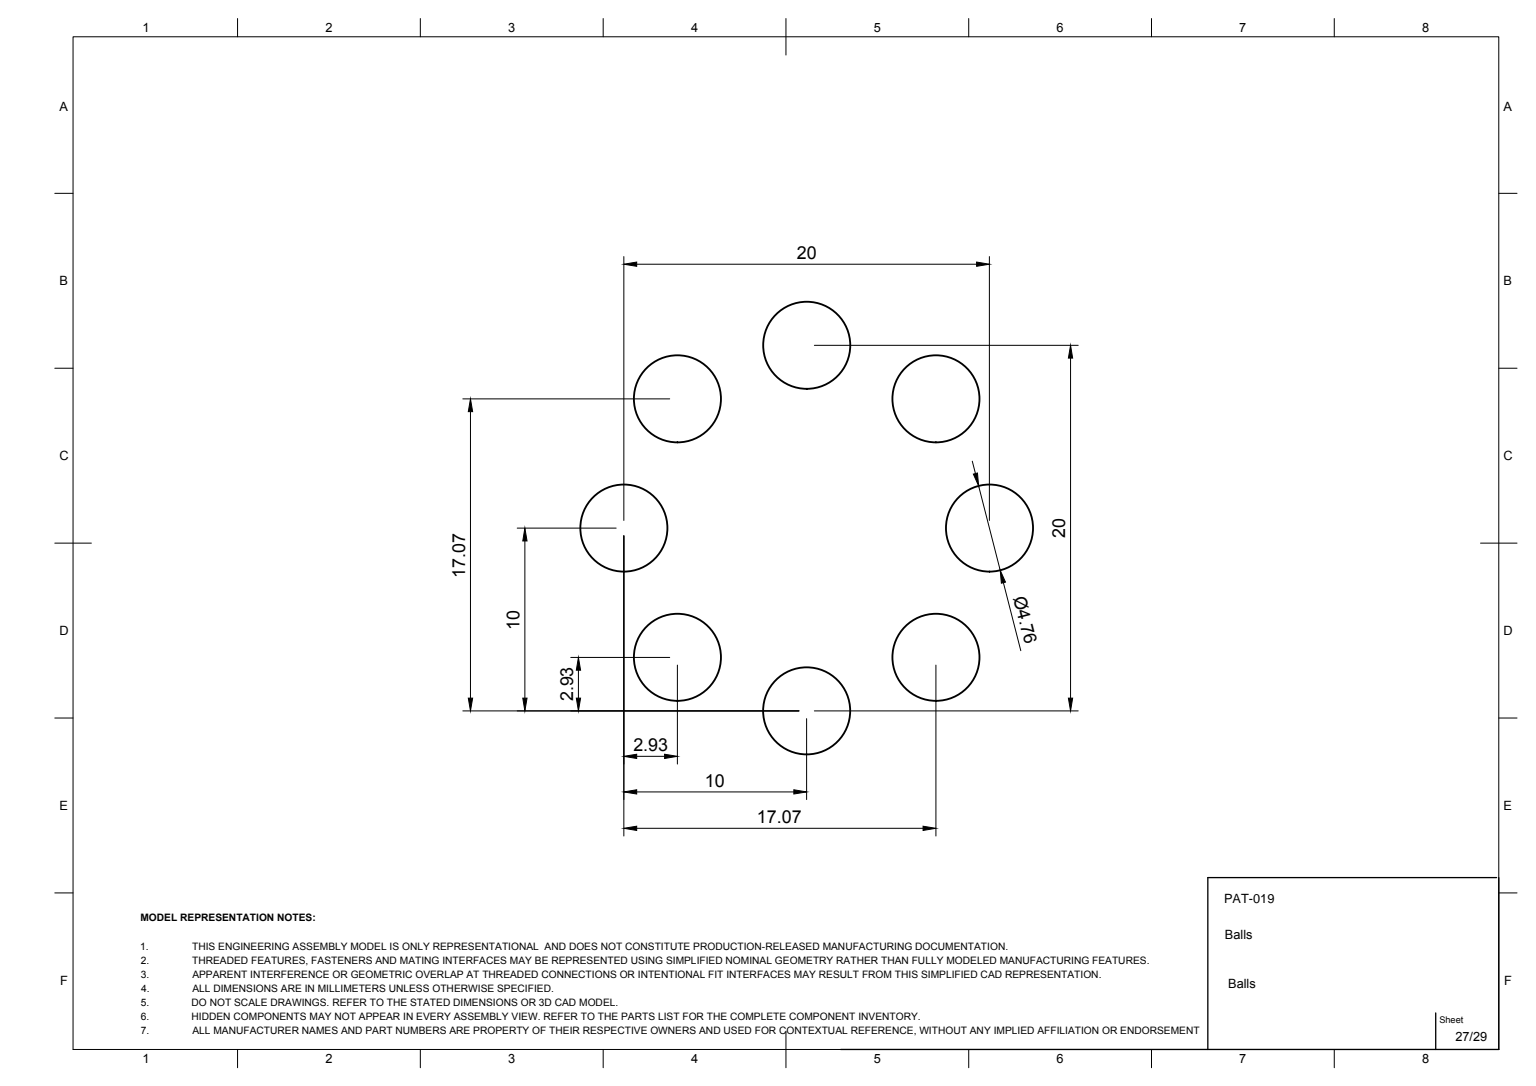
ISO-10303-21;
HEADER;
/* Generated by software containing ST-Developer
 * from STEP Tools, Inc. (www.steptools.com) 
 */

FILE_DESCRIPTION(
/* description */ ('Caster wheel assembly'),
/* implementation_level */ '2;1');

FILE_NAME(
/* name */ 'Balls.step',
/* time_stamp */ '2026-10-28T03:23:56-07:00',
/* author */ (''),
/* organization */ (''),
/* preprocessor_version */ 'ST-DEVELOPER v20.2',
/* originating_system */ 'Autodesk Translation Framework v15.17.0.0',
/* authorisation */ '');

FILE_SCHEMA (('AUTOMOTIVE_DESIGN { 1 0 10303 214 3 1 1 }'));
ENDSEC;

DATA;
#10=MECHANICAL_DESIGN_GEOMETRIC_PRESENTATION_REPRESENTATION('',(#241,#242,#243,#244,#245,#246,#247,#248),#5385);
#29=SPHERICAL_SURFACE('',#3204,0.23815);
#30=SPHERICAL_SURFACE('',#3206,0.23815);
#31=SPHERICAL_SURFACE('',#3208,0.23815);
#32=SPHERICAL_SURFACE('',#3210,0.23815);
#33=SPHERICAL_SURFACE('',#3212,0.23815);
#34=SPHERICAL_SURFACE('',#3214,0.23815);
#35=SPHERICAL_SURFACE('',#3216,0.23815);
#36=SPHERICAL_SURFACE('',#3218,0.23815);
#197=SHAPE_REPRESENTATION_RELATIONSHIP('SRR','None',#5495,#219);
#219=ADVANCED_BREP_SHAPE_REPRESENTATION('',(#270,#271,#272,#273,#274,#275,
#276,#277),#5382);
#241=STYLED_ITEM('',(#5672),#270);
#242=STYLED_ITEM('',(#5672),#271);
#243=STYLED_ITEM('',(#5672),#272);
#244=STYLED_ITEM('',(#5672),#273);
#245=STYLED_ITEM('',(#5672),#274);
#246=STYLED_ITEM('',(#5672),#275);
#247=STYLED_ITEM('',(#5672),#276);
#248=STYLED_ITEM('',(#5672),#277);
#270=MANIFOLD_SOLID_BREP('Body1',#2669);
#271=MANIFOLD_SOLID_BREP('Body2',#2670);
#272=MANIFOLD_SOLID_BREP('Body3',#2671);
#273=MANIFOLD_SOLID_BREP('Body4',#2672);
#274=MANIFOLD_SOLID_BREP('Body5',#2673);
#275=MANIFOLD_SOLID_BREP('Body6',#2674);
#276=MANIFOLD_SOLID_BREP('Body7',#2675);
#277=MANIFOLD_SOLID_BREP('Body8',#2676);
#554=FACE_OUTER_BOUND('',#769,.T.);
#555=FACE_OUTER_BOUND('',#770,.T.);
#556=FACE_OUTER_BOUND('',#771,.T.);
#557=FACE_OUTER_BOUND('',#772,.T.);
#558=FACE_OUTER_BOUND('',#773,.T.);
#559=FACE_OUTER_BOUND('',#774,.T.);
#560=FACE_OUTER_BOUND('',#775,.T.);
#561=FACE_OUTER_BOUND('',#776,.T.);
#769=EDGE_LOOP('',(#2280,#2281));
#770=EDGE_LOOP('',(#2282,#2283));
#771=EDGE_LOOP('',(#2284,#2285));
#772=EDGE_LOOP('',(#2286,#2287));
#773=EDGE_LOOP('',(#2288,#2289));
#774=EDGE_LOOP('',(#2290,#2291));
#775=EDGE_LOOP('',(#2292,#2293));
#776=EDGE_LOOP('',(#2294,#2295));
#1186=CIRCLE('',#3205,0.23815);
#1187=CIRCLE('',#3207,0.23815);
#1188=CIRCLE('',#3209,0.23815);
#1189=CIRCLE('',#3211,0.23815);
#1190=CIRCLE('',#3213,0.23815);
#1191=CIRCLE('',#3215,0.23815);
#1192=CIRCLE('',#3217,0.23815);
#1193=CIRCLE('',#3219,0.23815);
#1399=VERTEX_POINT('',#4809);
#1400=VERTEX_POINT('',#4810);
#1401=VERTEX_POINT('',#4813);
#1402=VERTEX_POINT('',#4814);
#1403=VERTEX_POINT('',#4817);
#1404=VERTEX_POINT('',#4818);
#1405=VERTEX_POINT('',#4821);
#1406=VERTEX_POINT('',#4822);
#1407=VERTEX_POINT('',#4825);
#1408=VERTEX_POINT('',#4826);
#1409=VERTEX_POINT('',#4829);
#1410=VERTEX_POINT('',#4830);
#1411=VERTEX_POINT('',#4833);
#1412=VERTEX_POINT('',#4834);
#1413=VERTEX_POINT('',#4837);
#1414=VERTEX_POINT('',#4838);
#1708=EDGE_CURVE('',#1399,#1400,#1186,.T.);
#1709=EDGE_CURVE('',#1401,#1402,#1187,.T.);
#1710=EDGE_CURVE('',#1403,#1404,#1188,.T.);
#1711=EDGE_CURVE('',#1405,#1406,#1189,.T.);
#1712=EDGE_CURVE('',#1407,#1408,#1190,.T.);
#1713=EDGE_CURVE('',#1409,#1410,#1191,.T.);
#1714=EDGE_CURVE('',#1411,#1412,#1192,.T.);
#1715=EDGE_CURVE('',#1413,#1414,#1193,.T.);
#2280=ORIENTED_EDGE('',*,*,#1708,.T.);
#2281=ORIENTED_EDGE('',*,*,#1708,.F.);
#2282=ORIENTED_EDGE('',*,*,#1709,.T.);
#2283=ORIENTED_EDGE('',*,*,#1709,.F.);
#2284=ORIENTED_EDGE('',*,*,#1710,.T.);
#2285=ORIENTED_EDGE('',*,*,#1710,.F.);
#2286=ORIENTED_EDGE('',*,*,#1711,.T.);
#2287=ORIENTED_EDGE('',*,*,#1711,.F.);
#2288=ORIENTED_EDGE('',*,*,#1712,.T.);
#2289=ORIENTED_EDGE('',*,*,#1712,.F.);
#2290=ORIENTED_EDGE('',*,*,#1713,.T.);
#2291=ORIENTED_EDGE('',*,*,#1713,.F.);
#2292=ORIENTED_EDGE('',*,*,#1714,.T.);
#2293=ORIENTED_EDGE('',*,*,#1714,.F.);
#2294=ORIENTED_EDGE('',*,*,#1715,.T.);
#2295=ORIENTED_EDGE('',*,*,#1715,.F.);
#2614=ADVANCED_FACE('',(#554),#29,.T.);
#2615=ADVANCED_FACE('',(#555),#30,.T.);
#2616=ADVANCED_FACE('',(#556),#31,.T.);
#2617=ADVANCED_FACE('',(#557),#32,.T.);
#2618=ADVANCED_FACE('',(#558),#33,.T.);
#2619=ADVANCED_FACE('',(#559),#34,.T.);
#2620=ADVANCED_FACE('',(#560),#35,.T.);
#2621=ADVANCED_FACE('',(#561),#36,.T.);
#2669=CLOSED_SHELL('',(#2614));
#2670=CLOSED_SHELL('',(#2615));
#2671=CLOSED_SHELL('',(#2616));
#2672=CLOSED_SHELL('',(#2617));
#2673=CLOSED_SHELL('',(#2618));
#2674=CLOSED_SHELL('',(#2619));
#2675=CLOSED_SHELL('',(#2620));
#2676=CLOSED_SHELL('',(#2621));
#3203=AXIS2_PLACEMENT_3D('',#4807,#3992,#3993);
#3204=AXIS2_PLACEMENT_3D('',#4808,#3994,#3995);
#3205=AXIS2_PLACEMENT_3D('',#4811,#3996,#3997);
#3206=AXIS2_PLACEMENT_3D('',#4812,#3998,#3999);
#3207=AXIS2_PLACEMENT_3D('',#4815,#4000,#4001);
#3208=AXIS2_PLACEMENT_3D('',#4816,#4002,#4003);
#3209=AXIS2_PLACEMENT_3D('',#4819,#4004,#4005);
#3210=AXIS2_PLACEMENT_3D('',#4820,#4006,#4007);
#3211=AXIS2_PLACEMENT_3D('',#4823,#4008,#4009);
#3212=AXIS2_PLACEMENT_3D('',#4824,#4010,#4011);
#3213=AXIS2_PLACEMENT_3D('',#4827,#4012,#4013);
#3214=AXIS2_PLACEMENT_3D('',#4828,#4014,#4015);
#3215=AXIS2_PLACEMENT_3D('',#4831,#4016,#4017);
#3216=AXIS2_PLACEMENT_3D('',#4832,#4018,#4019);
#3217=AXIS2_PLACEMENT_3D('',#4835,#4020,#4021);
#3218=AXIS2_PLACEMENT_3D('',#4836,#4022,#4023);
#3219=AXIS2_PLACEMENT_3D('',#4839,#4024,#4025);
#3992=DIRECTION('axis',(0.,0.,1.));
#3993=DIRECTION('refdir',(1.,0.,0.));
#3994=DIRECTION('center_axis',(0.,0.,1.));
#3995=DIRECTION('ref_axis',(1.,0.,0.));
#3996=DIRECTION('center_axis',(1.22464679914735E-16,-1.,0.));
#3997=DIRECTION('ref_axis',(-1.,-1.22464679914735E-16,0.));
#3998=DIRECTION('center_axis',(0.707106781186548,0.,0.707106781186548));
#3999=DIRECTION('ref_axis',(0.707106781186548,0.,-0.707106781186548));
#4000=DIRECTION('center_axis',(8.65956056235494E-17,-1.,-8.65956056235493E-17));
#4001=DIRECTION('ref_axis',(-0.707106781186547,-1.22464679914735E-16,0.707106781186547));
#4002=DIRECTION('center_axis',(1.,0.,0.));
#4003=DIRECTION('ref_axis',(6.12323399573676E-17,0.,-1.));
#4004=DIRECTION('center_axis',(7.49879891330929E-33,-1.,-1.22464679914735E-16));
#4005=DIRECTION('ref_axis',(-6.12323399573676E-17,-1.22464679914735E-16,
1.));
#4006=DIRECTION('center_axis',(0.707106781186548,0.,-0.707106781186548));
#4007=DIRECTION('ref_axis',(-0.707106781186548,0.,-0.707106781186548));
#4008=DIRECTION('center_axis',(-8.65956056235493E-17,-1.,-8.65956056235494E-17));
#4009=DIRECTION('ref_axis',(0.707106781186547,-1.22464679914735E-16,0.707106781186547));
#4010=DIRECTION('center_axis',(0.,0.,-1.));
#4011=DIRECTION('ref_axis',(-1.,0.,-1.22464679914735E-16));
#4012=DIRECTION('center_axis',(-1.22464679914735E-16,-1.,-1.49975978266186E-32));
#4013=DIRECTION('ref_axis',(1.,-1.22464679914735E-16,1.22464679914735E-16));
#4014=DIRECTION('center_axis',(-0.707106781186547,0.,-0.707106781186548));
#4015=DIRECTION('ref_axis',(-0.707106781186548,0.,0.707106781186547));
#4016=DIRECTION('center_axis',(-8.65956056235493E-17,-1.,8.65956056235493E-17));
#4017=DIRECTION('ref_axis',(0.707106781186548,-1.22464679914735E-16,-0.707106781186547));
#4018=DIRECTION('center_axis',(-1.,0.,0.));
#4019=DIRECTION('ref_axis',(-1.83697019872103E-16,0.,1.));
#4020=DIRECTION('center_axis',(-2.24963967399279E-32,-1.,1.22464679914735E-16));
#4021=DIRECTION('ref_axis',(1.83697019872103E-16,-1.22464679914735E-16,
-1.));
#4022=DIRECTION('center_axis',(-0.707106781186548,0.,0.707106781186548));
#4023=DIRECTION('ref_axis',(0.707106781186547,0.,0.707106781186548));
#4024=DIRECTION('center_axis',(8.65956056235493E-17,-1.,8.65956056235493E-17));
#4025=DIRECTION('ref_axis',(-0.707106781186547,-1.22464679914735E-16,-0.707106781186548));
#4807=CARTESIAN_POINT('',(0.,0.,0.));
#4808=CARTESIAN_POINT('Origin',(1.,0.,0.));
#4809=CARTESIAN_POINT('',(1.,-1.78583896120461E-33,0.23815));
#4810=CARTESIAN_POINT('',(1.,-1.78583896120461E-33,-0.23815));
#4811=CARTESIAN_POINT('Origin',(1.,0.,0.));
#4812=CARTESIAN_POINT('Origin',(0.707106781186548,0.,-0.707106781186547));
#4813=CARTESIAN_POINT('',(0.875504261126124,-1.78583896120461E-33,-0.538709301246971));
#4814=CARTESIAN_POINT('',(0.538709301246971,-1.78583896120461E-33,-0.875504261126124));
#4815=CARTESIAN_POINT('Origin',(0.707106781186548,0.,-0.707106781186547));
#4816=CARTESIAN_POINT('Origin',(6.12323399573677E-17,0.,-1.));
#4817=CARTESIAN_POINT('',(0.23815,-1.78583896120461E-33,-1.));
#4818=CARTESIAN_POINT('',(-0.23815,-1.78583896120461E-33,-1.));
#4819=CARTESIAN_POINT('Origin',(6.12323399573677E-17,0.,-1.));
#4820=CARTESIAN_POINT('Origin',(-0.707106781186547,0.,-0.707106781186548));
#4821=CARTESIAN_POINT('',(-0.538709301246971,-1.78583896120461E-33,-0.875504261126124));
#4822=CARTESIAN_POINT('',(-0.875504261126124,-1.78583896120461E-33,-0.538709301246971));
#4823=CARTESIAN_POINT('Origin',(-0.707106781186547,0.,-0.707106781186548));
#4824=CARTESIAN_POINT('Origin',(-1.,0.,-1.22464679914735E-16));
#4825=CARTESIAN_POINT('',(-1.,-1.78583896120461E-33,-0.23815));
#4826=CARTESIAN_POINT('',(-1.,-1.78583896120461E-33,0.23815));
#4827=CARTESIAN_POINT('Origin',(-1.,0.,-1.22464679914735E-16));
#4828=CARTESIAN_POINT('Origin',(-0.707106781186548,0.,0.707106781186547));
#4829=CARTESIAN_POINT('',(-0.875504261126124,-7.94881478324376E-33,0.538709301246971));
#4830=CARTESIAN_POINT('',(-0.538709301246971,4.37713686083455E-33,0.875504261126124));
#4831=CARTESIAN_POINT('Origin',(-0.707106781186548,0.,0.707106781186547));
#4832=CARTESIAN_POINT('Origin',(-1.83697019872103E-16,0.,1.));
#4833=CARTESIAN_POINT('',(-0.23815,-1.78583896120461E-33,1.));
#4834=CARTESIAN_POINT('',(0.23815,-1.78583896120461E-33,1.));
#4835=CARTESIAN_POINT('Origin',(-1.83697019872103E-16,0.,1.));
#4836=CARTESIAN_POINT('Origin',(0.707106781186547,0.,0.707106781186548));
#4837=CARTESIAN_POINT('',(0.538709301246971,-4.86732687222419E-33,0.875504261126124));
#4838=CARTESIAN_POINT('',(0.875504261126124,1.29564894981497E-33,0.538709301246971));
#4839=CARTESIAN_POINT('Origin',(0.707106781186547,0.,0.707106781186548));
#5354=UNCERTAINTY_MEASURE_WITH_UNIT(LENGTH_MEASURE(0.001),#5386,
'DISTANCE_ACCURACY_VALUE',
'Maximum model space distance between geometric entities at asserted c
onnectivities');
#5357=UNCERTAINTY_MEASURE_WITH_UNIT(LENGTH_MEASURE(0.001),#5386,
'DISTANCE_ACCURACY_VALUE',
'Maximum model space distance between geometric entities at asserted c
onnectivities');
#5382=(
GEOMETRIC_REPRESENTATION_CONTEXT(3)
GLOBAL_UNCERTAINTY_ASSIGNED_CONTEXT((#5354))
GLOBAL_UNIT_ASSIGNED_CONTEXT((#5386,#5388,#5389))
REPRESENTATION_CONTEXT('','3D')
);
#5385=(
GEOMETRIC_REPRESENTATION_CONTEXT(3)
GLOBAL_UNCERTAINTY_ASSIGNED_CONTEXT((#5357))
GLOBAL_UNIT_ASSIGNED_CONTEXT((#5386,#5388,#5389))
REPRESENTATION_CONTEXT('','3D')
);
#5386=(
LENGTH_UNIT()
NAMED_UNIT(*)
SI_UNIT(.CENTI.,.METRE.)
);
#5388=(
NAMED_UNIT(*)
PLANE_ANGLE_UNIT()
SI_UNIT($,.RADIAN.)
);
#5389=(
NAMED_UNIT(*)
SI_UNIT($,.STERADIAN.)
SOLID_ANGLE_UNIT()
);
#5414=SHAPE_DEFINITION_REPRESENTATION(#5455,#5495);
#5455=PRODUCT_DEFINITION_SHAPE('',$,#5523);
#5495=SHAPE_REPRESENTATION('',(#3203),#5382);
#5498=PRODUCT_DEFINITION_CONTEXT('part definition',#5581,'design');
#5523=PRODUCT_DEFINITION('Balls','Balls',#5550,#5498);
#5550=PRODUCT_DEFINITION_FORMATION('',$,#5607);
#5581=APPLICATION_CONTEXT(
'Core Data for Automotive Mechanical Design Process');
#5582=PRODUCT_CONTEXT('part definition',#5581,'mechanical');
#5607=PRODUCT('Balls','Balls','Balls',(#5582));
#5666=COLOUR_RGB('Grey',0.48,0.52,0.57);
#5667=FILL_AREA_STYLE_COLOUR('',#5666);
#5668=FILL_AREA_STYLE('',(#5667));
#5669=SURFACE_STYLE_FILL_AREA(#5668);
#5670=SURFACE_SIDE_STYLE('',(#5669));
#5671=SURFACE_STYLE_USAGE(.BOTH.,#5670);
#5672=PRESENTATION_STYLE_ASSIGNMENT((#5671));
ENDSEC;
END-ISO-10303-21;
